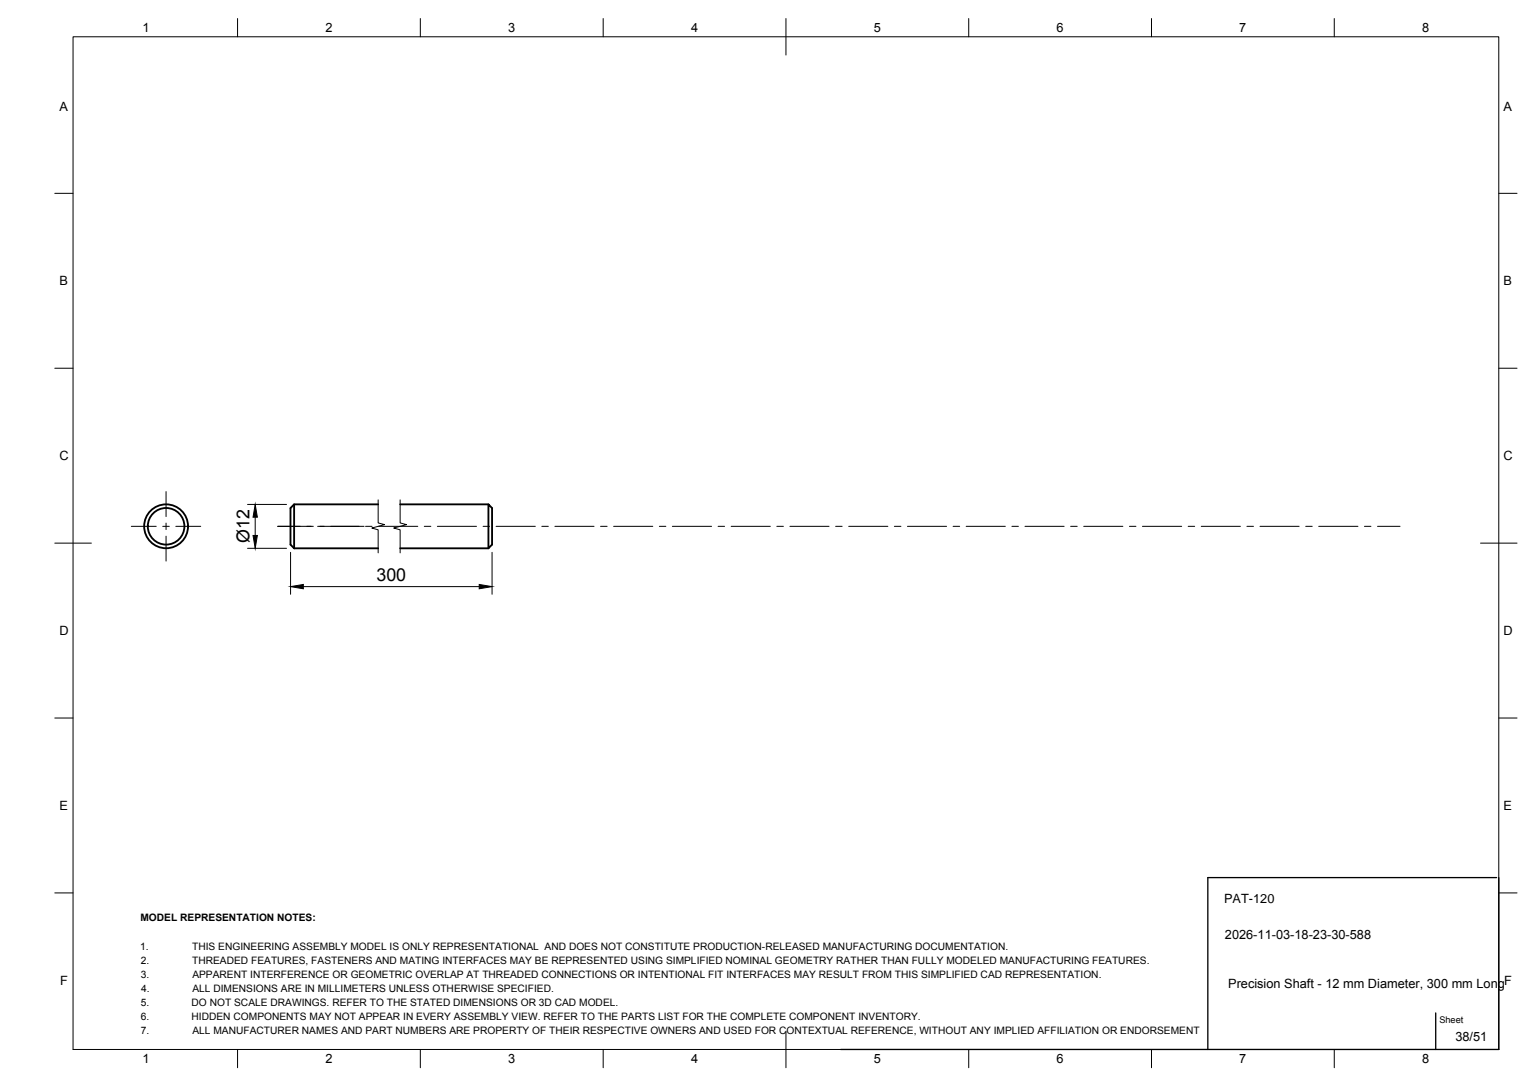
ISO-10303-21;
HEADER;
/* Generated by software containing ST-Developer
 * from STEP Tools, Inc. (www.steptools.com) 
 */

FILE_DESCRIPTION(
/* description */ ('Vibration shaker table dummy'),
/* implementation_level */ '2;1');

FILE_NAME(
/* name */ 'Precision Shaft - 12 mm Diameter, 300 mm Long.step',
/* time_stamp */ '2026-10-27T10:55:14-07:00',
/* author */ (''),
/* organization */ (''),
/* preprocessor_version */ 'ST-DEVELOPER v20.2',
/* originating_system */ 'Autodesk Translation Framework v15.17.0.0',
/* authorisation */ '');

FILE_SCHEMA (('AUTOMOTIVE_DESIGN { 1 0 10303 214 3 1 1 }'));
ENDSEC;

DATA;
#10=MECHANICAL_DESIGN_GEOMETRIC_PRESENTATION_REPRESENTATION('',(#719),#22394);
#573=CONICAL_SURFACE('',#10340,0.55,0.785398163397448);
#574=CONICAL_SURFACE('',#10346,0.55,0.785398163397441);
#627=SHAPE_REPRESENTATION_RELATIONSHIP('SRR','None',#22673,#673);
#673=ADVANCED_BREP_SHAPE_REPRESENTATION('',(#765),#22379);
#719=STYLED_ITEM('',(#22961),#765);
#765=MANIFOLD_SOLID_BREP('Body1',#9237);
#1232=PLANE('',#10345);
#1233=PLANE('',#10348);
#1633=FACE_OUTER_BOUND('',#2303,.T.);
#1634=FACE_OUTER_BOUND('',#2304,.T.);
#1635=FACE_OUTER_BOUND('',#2305,.T.);
#1636=FACE_OUTER_BOUND('',#2306,.T.);
#1637=FACE_OUTER_BOUND('',#2307,.T.);
#2303=EDGE_LOOP('',(#7494,#7495,#7496,#7497));
#2304=EDGE_LOOP('',(#7498,#7499,#7500,#7501));
#2305=EDGE_LOOP('',(#7502));
#2306=EDGE_LOOP('',(#7503,#7504,#7505,#7506));
#2307=EDGE_LOOP('',(#7507));
#2986=LINE('',#21099,#3605);
#2987=LINE('',#21104,#3606);
#2988=LINE('',#21109,#3607);
#3605=VECTOR('',#12478,0.55);
#3606=VECTOR('',#12485,0.6);
#3607=VECTOR('',#12492,0.55);
#4116=CIRCLE('',#10341,0.6);
#4117=CIRCLE('',#10342,0.5);
#4118=CIRCLE('',#10344,0.6);
#4119=CIRCLE('',#10347,0.5);
#4783=VERTEX_POINT('',#21096);
#4784=VERTEX_POINT('',#21098);
#4785=VERTEX_POINT('',#21102);
#4786=VERTEX_POINT('',#21107);
#5740=EDGE_CURVE('',#4783,#4783,#4116,.T.);
#5741=EDGE_CURVE('',#4783,#4784,#2986,.T.);
#5742=EDGE_CURVE('',#4784,#4784,#4117,.T.);
#5743=EDGE_CURVE('',#4785,#4785,#4118,.T.);
#5744=EDGE_CURVE('',#4785,#4783,#2987,.T.);
#5745=EDGE_CURVE('',#4786,#4786,#4119,.T.);
#5746=EDGE_CURVE('',#4786,#4785,#2988,.T.);
#7494=ORIENTED_EDGE('',*,*,#5740,.T.);
#7495=ORIENTED_EDGE('',*,*,#5741,.T.);
#7496=ORIENTED_EDGE('',*,*,#5742,.T.);
#7497=ORIENTED_EDGE('',*,*,#5741,.F.);
#7498=ORIENTED_EDGE('',*,*,#5743,.F.);
#7499=ORIENTED_EDGE('',*,*,#5744,.T.);
#7500=ORIENTED_EDGE('',*,*,#5740,.F.);
#7501=ORIENTED_EDGE('',*,*,#5744,.F.);
#7502=ORIENTED_EDGE('',*,*,#5742,.F.);
#7503=ORIENTED_EDGE('',*,*,#5745,.T.);
#7504=ORIENTED_EDGE('',*,*,#5746,.T.);
#7505=ORIENTED_EDGE('',*,*,#5743,.T.);
#7506=ORIENTED_EDGE('',*,*,#5746,.F.);
#7507=ORIENTED_EDGE('',*,*,#5745,.F.);
#8622=CYLINDRICAL_SURFACE('',#10343,0.6);
#8998=ADVANCED_FACE('',(#1633),#573,.T.);
#8999=ADVANCED_FACE('',(#1634),#8622,.T.);
#9000=ADVANCED_FACE('',(#1635),#1232,.F.);
#9001=ADVANCED_FACE('',(#1636),#574,.T.);
#9002=ADVANCED_FACE('',(#1637),#1233,.T.);
#9237=CLOSED_SHELL('',(#8998,#8999,#9000,#9001,#9002));
#10339=AXIS2_PLACEMENT_3D('',#21094,#12472,#12473);
#10340=AXIS2_PLACEMENT_3D('',#21095,#12474,#12475);
#10341=AXIS2_PLACEMENT_3D('',#21097,#12476,#12477);
#10342=AXIS2_PLACEMENT_3D('',#21100,#12479,#12480);
#10343=AXIS2_PLACEMENT_3D('',#21101,#12481,#12482);
#10344=AXIS2_PLACEMENT_3D('',#21103,#12483,#12484);
#10345=AXIS2_PLACEMENT_3D('',#21105,#12486,#12487);
#10346=AXIS2_PLACEMENT_3D('',#21106,#12488,#12489);
#10347=AXIS2_PLACEMENT_3D('',#21108,#12490,#12491);
#10348=AXIS2_PLACEMENT_3D('',#21110,#12493,#12494);
#12472=DIRECTION('axis',(0.,0.,1.));
#12473=DIRECTION('refdir',(1.,0.,0.));
#12474=DIRECTION('center_axis',(1.,0.,0.));
#12475=DIRECTION('ref_axis',(0.,0.,-1.));
#12476=DIRECTION('center_axis',(-1.,0.,0.));
#12477=DIRECTION('ref_axis',(0.,0.,-1.));
#12478=DIRECTION('',(-0.707106781186548,8.65956056235493E-17,-0.707106781186547));
#12479=DIRECTION('center_axis',(1.,0.,0.));
#12480=DIRECTION('ref_axis',(0.,0.,-1.));
#12481=DIRECTION('center_axis',(1.,0.,0.));
#12482=DIRECTION('ref_axis',(0.,0.,-1.));
#12483=DIRECTION('center_axis',(1.,0.,0.));
#12484=DIRECTION('ref_axis',(0.,0.,-1.));
#12485=DIRECTION('',(-1.,0.,0.));
#12486=DIRECTION('center_axis',(1.,0.,0.));
#12487=DIRECTION('ref_axis',(0.,0.,-1.));
#12488=DIRECTION('center_axis',(-1.,0.,0.));
#12489=DIRECTION('ref_axis',(0.,0.,-1.));
#12490=DIRECTION('center_axis',(-1.,0.,0.));
#12491=DIRECTION('ref_axis',(0.,0.,-1.));
#12492=DIRECTION('',(-0.707106781186553,-8.65956056235487E-17,0.707106781186542));
#12493=DIRECTION('center_axis',(1.,0.,0.));
#12494=DIRECTION('ref_axis',(0.,0.,-1.));
#21094=CARTESIAN_POINT('',(0.,0.,0.));
#21095=CARTESIAN_POINT('Origin',(0.05,0.,0.));
#21096=CARTESIAN_POINT('',(0.1,7.34788079488412E-17,0.6));
#21097=CARTESIAN_POINT('Origin',(0.1,0.,0.));
#21098=CARTESIAN_POINT('',(0.,-6.12323399573677E-17,0.5));
#21099=CARTESIAN_POINT('',(0.05,-6.73555739531044E-17,0.55));
#21100=CARTESIAN_POINT('Origin',(0.,0.,0.));
#21101=CARTESIAN_POINT('Origin',(0.,0.,0.));
#21102=CARTESIAN_POINT('',(29.9,-7.34788079488412E-17,0.6));
#21103=CARTESIAN_POINT('Origin',(29.9,0.,0.));
#21104=CARTESIAN_POINT('',(0.,-7.34788079488412E-17,0.6));
#21105=CARTESIAN_POINT('Origin',(0.,0.,0.));
#21106=CARTESIAN_POINT('Origin',(29.95,0.,0.));
#21107=CARTESIAN_POINT('',(30.,6.12323399573677E-17,0.5));
#21108=CARTESIAN_POINT('Origin',(30.,0.,0.));
#21109=CARTESIAN_POINT('',(29.95,-6.73555739531044E-17,0.55));
#21110=CARTESIAN_POINT('Origin',(30.,0.,0.));
#22328=UNCERTAINTY_MEASURE_WITH_UNIT(LENGTH_MEASURE(0.001),#22395,
'DISTANCE_ACCURACY_VALUE',
'Maximum model space distance between geometric entities at asserted c
onnectivities');
#22343=UNCERTAINTY_MEASURE_WITH_UNIT(LENGTH_MEASURE(0.001),#22395,
'DISTANCE_ACCURACY_VALUE',
'Maximum model space distance between geometric entities at asserted c
onnectivities');
#22379=(
GEOMETRIC_REPRESENTATION_CONTEXT(3)
GLOBAL_UNCERTAINTY_ASSIGNED_CONTEXT((#22328))
GLOBAL_UNIT_ASSIGNED_CONTEXT((#22395,#22397,#22398))
REPRESENTATION_CONTEXT('','3D')
);
#22394=(
GEOMETRIC_REPRESENTATION_CONTEXT(3)
GLOBAL_UNCERTAINTY_ASSIGNED_CONTEXT((#22343))
GLOBAL_UNIT_ASSIGNED_CONTEXT((#22395,#22397,#22398))
REPRESENTATION_CONTEXT('','3D')
);
#22395=(
LENGTH_UNIT()
NAMED_UNIT(*)
SI_UNIT(.CENTI.,.METRE.)
);
#22397=(
NAMED_UNIT(*)
PLANE_ANGLE_UNIT()
SI_UNIT($,.RADIAN.)
);
#22398=(
NAMED_UNIT(*)
SI_UNIT($,.STERADIAN.)
SOLID_ANGLE_UNIT()
);
#22434=SHAPE_DEFINITION_REPRESENTATION(#22484,#22673);
#22484=PRODUCT_DEFINITION_SHAPE('',$,#22724);
#22673=SHAPE_REPRESENTATION('',(#10339),#22379);
#22688=PRODUCT_DEFINITION_CONTEXT('part definition',#22840,'design');
#22724=PRODUCT_DEFINITION(
'Precision Shaft - 12 mm Diameter, 300 mm Long',
'Precision Shaft - 12 mm Diameter, 300 mm Long',#22774,#22688);
#22774=PRODUCT_DEFINITION_FORMATION('',$,#22877);
#22840=APPLICATION_CONTEXT(
'Core Data for Automotive Mechanical Design Process');
#22841=PRODUCT_CONTEXT('part definition',#22840,'mechanical');
#22877=PRODUCT('Precision Shaft - 12 mm Diameter, 300 mm Long',
'Precision Shaft - 12 mm Diameter, 300 mm Long',
'Precision Shaft - 12 mm Diameter, 300 mm Long',(#22841));
#22955=COLOUR_RGB('Grey',0.48,0.52,0.57);
#22956=FILL_AREA_STYLE_COLOUR('',#22955);
#22957=FILL_AREA_STYLE('',(#22956));
#22958=SURFACE_STYLE_FILL_AREA(#22957);
#22959=SURFACE_SIDE_STYLE('',(#22958));
#22960=SURFACE_STYLE_USAGE(.BOTH.,#22959);
#22961=PRESENTATION_STYLE_ASSIGNMENT((#22960));
ENDSEC;
END-ISO-10303-21;
